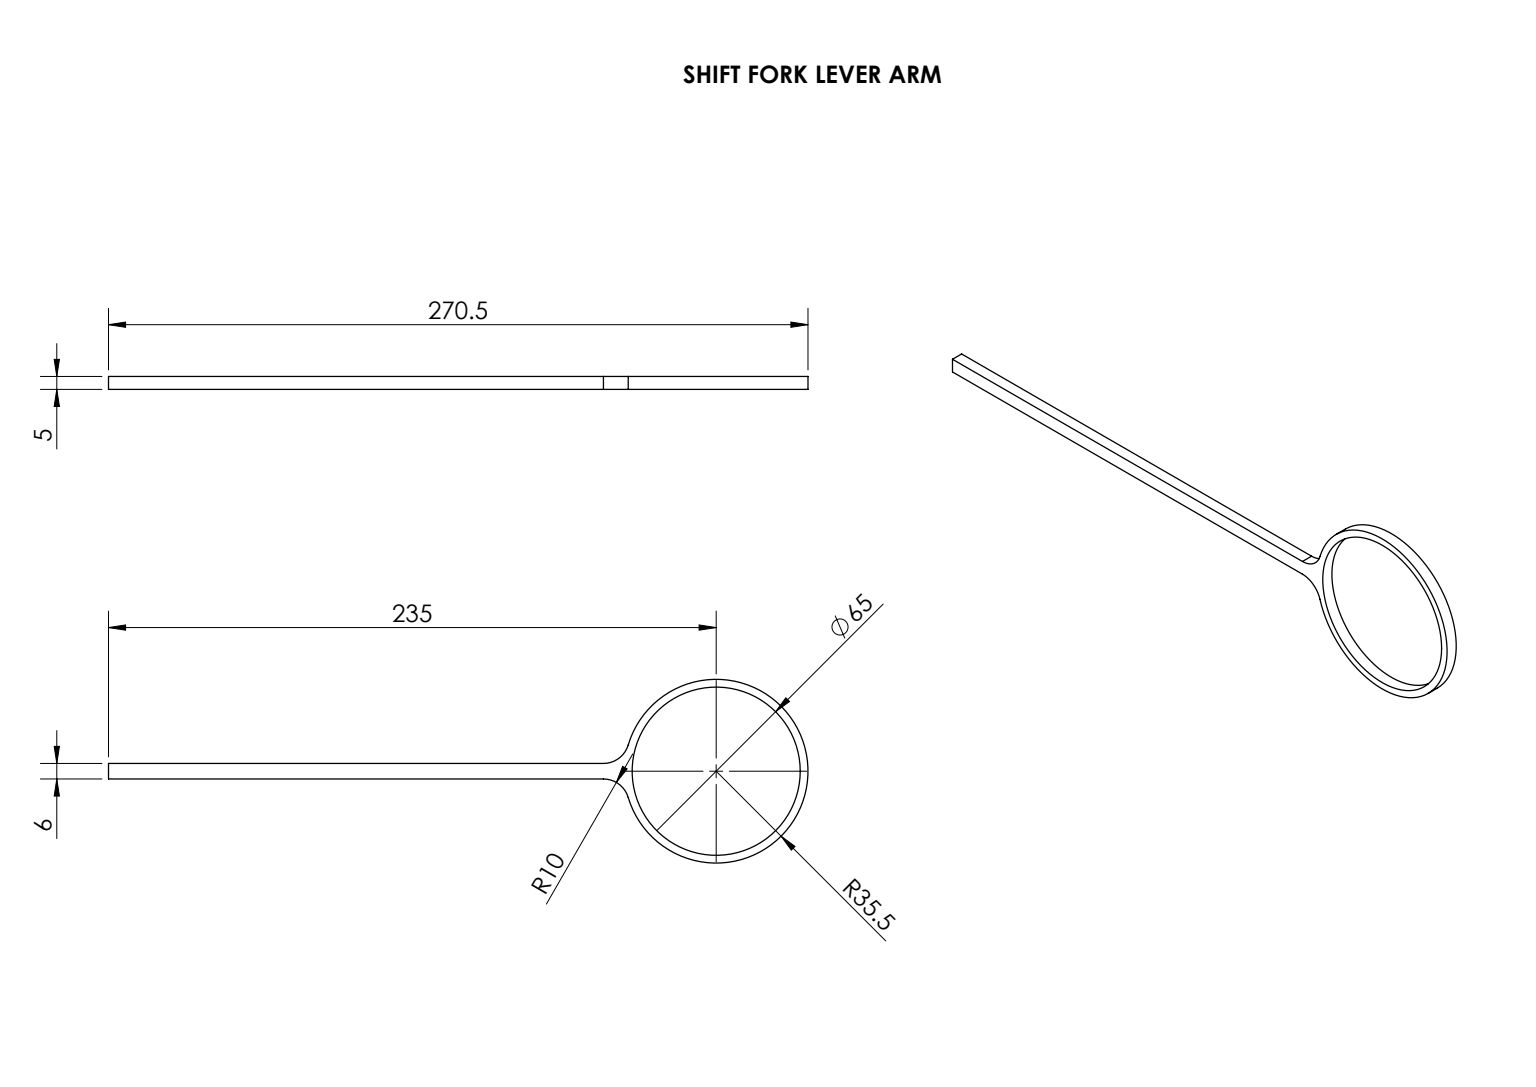
ISO-10303-21;
HEADER;
FILE_DESCRIPTION (('STEP AP214'),
    '1' );
FILE_NAME ('Shift Fork Lever Arm.step',
    '2026-09-30T12:41:04',
    ( '' ),
    ( '' ),
    'SwSTEP 2.0',
    'SolidWorks 2026',
    '' );
FILE_SCHEMA (( 'AUTOMOTIVE_DESIGN' ));
ENDSEC;

DATA;
#251=EDGE_CURVE ( 'NONE', #37160, #31484, #24741, .T. ) ;
#287=AXIS2_PLACEMENT_3D ( 'NONE', #20110, #9559, #24504 ) ;
#332=LINE ( 'NONE', #22378, #45772 ) ;
#605=ADVANCED_BREP_SHAPE_REPRESENTATION ( '', ( #3244, #11636 ), #6986 ) ;
#623=DIRECTION ( 'NONE',  ( 0.000000000000000000, 0.000000000000000000, 1.000000000000000000 ) ) ;
#1121=PRODUCT_DEFINITION ( 'UNKNOWN', '', #32690, #14935 ) ;
#1167=DIRECTION ( 'NONE',  ( 1.000000000000000000, 0.000000000000000000, 0.000000000000000000 ) ) ;
#1414=ORIENTED_EDGE ( 'NONE', *, *, #47268, .F. ) ;
#1530=EDGE_CURVE ( 'NONE', #31484, #24326, #4202, .T. ) ;
#1531=CARTESIAN_POINT ( 'NONE',  ( -43.60332556124591719, -117.0000000000000000, -2.500000000000002220 ) ) ;
#1603=ORIENTED_EDGE ( 'NONE', *, *, #35461, .T. ) ;
#1694=FILL_AREA_STYLE_COLOUR ( '', #30434 ) ;
#1768=VECTOR ( 'NONE', #29838, 1000.000000000000000 ) ;
#1821=EDGE_LOOP ( 'NONE', ( #25451, #11030, #4966, #38289 ) ) ;
#1945=( NAMED_UNIT ( * ) SI_UNIT ( $, .STERADIAN. ) SOLID_ANGLE_UNIT ( ) );
#2151=DIRECTION ( 'NONE',  ( -1.000000000000000000, 0.000000000000000000, 0.000000000000000000 ) ) ;
#2172=DIRECTION ( 'NONE',  ( 1.000000000000000000, 0.000000000000000000, 0.000000000000000000 ) ) ;
#2540=DIRECTION ( 'NONE',  ( 1.000000000000000000, 0.000000000000000000, 0.000000000000000000 ) ) ;
#2824=ADVANCED_FACE ( 'NONE', ( #8419 ), #23345, .F. ) ;
#2951=DIRECTION ( 'NONE',  ( 0.000000000000000000, 0.000000000000000000, 1.000000000000000000 ) ) ;
#3244=MANIFOLD_SOLID_BREP ( 'Fillet1', #6745 ) ;
#3247=VECTOR ( 'NONE', #47516, 1000.000000000000000 ) ;
#3362=ORIENTED_EDGE ( 'NONE', *, *, #41369, .F. ) ;
#3400=CARTESIAN_POINT ( 'NONE',  ( -235.0000123116479926, -117.0000000000000142, 2.500000000000000000 ) ) ;
#3500=ORIENTED_EDGE ( 'NONE', *, *, #6790, .F. ) ;
#3532=DIRECTION ( 'NONE',  ( -0.000000000000000000, -0.000000000000000000, -1.000000000000000000 ) ) ;
#3667=DIRECTION ( 'NONE',  ( 1.000000000000000000, 0.000000000000000000, 0.000000000000000000 ) ) ;
#3690=VERTEX_POINT ( 'NONE', #9677 ) ;
#3885=CARTESIAN_POINT ( 'NONE',  ( -43.60332556124591008, -133.0000000000000000, 2.500000000000002220 ) ) ;
#3916=FACE_OUTER_BOUND ( 'NONE', #19929, .T. ) ;
#4202=LINE ( 'NONE', #30155, #45519 ) ;
#4484=CARTESIAN_POINT ( 'NONE',  ( -35.37301231164799731, -117.0000000000000000, 2.500000000000000000 ) ) ;
#4520=ORIENTED_EDGE ( 'NONE', *, *, #32367, .F. ) ;
#4521=CARTESIAN_POINT ( 'NONE',  ( -35.37301231164799731, -123.0000000000000142, 2.500000000000000000 ) ) ;
#4650=VERTEX_POINT ( 'NONE', #6360 ) ;
#4684=FACE_BOUND ( 'NONE', #4938, .T. ) ;
#4787=ORIENTED_EDGE ( 'NONE', *, *, #19891, .F. ) ;
#4938=EDGE_LOOP ( 'NONE', ( #16511, #37210 ) ) ;
#4966=ORIENTED_EDGE ( 'NONE', *, *, #11266, .T. ) ;
#5358=( NAMED_UNIT ( * ) PLANE_ANGLE_UNIT ( ) SI_UNIT ( $, .RADIAN. ) );
#5684=ORIENTED_EDGE ( 'NONE', *, *, #1530, .F. ) ;
#5751=ORIENTED_EDGE ( 'NONE', *, *, #29832, .T. ) ;
#6138=FACE_OUTER_BOUND ( 'NONE', #42443, .T. ) ;
#6195=PRODUCT ( 'Shift Fork Lever Arm', 'Shift Fork Lever Arm', '', ( #34306 ) ) ;
#6360=CARTESIAN_POINT ( 'NONE',  ( -34.02017708624680381, -130.1428571428571388, 2.500000000000000000 ) ) ;
#6380=CARTESIAN_POINT ( 'NONE',  ( -235.0000123116479926, -123.0000000000000284, 2.500000000000000000 ) ) ;
#6513=ORIENTED_EDGE ( 'NONE', *, *, #11266, .F. ) ;
#6619=DIRECTION ( 'NONE',  ( 0.000000000000000000, 0.000000000000000000, 1.000000000000000000 ) ) ;
#6701=ADVANCED_FACE ( 'NONE', ( #47322 ), #17918, .F. ) ;
#6745=CLOSED_SHELL ( 'NONE', ( #35945, #26592, #34256, #14741, #7793, #6701, #7128, #14982, #2824, #10559 ) ) ;
#6790=EDGE_CURVE ( 'NONE', #4650, #23089, #28936, .T. ) ;
#6884=VERTEX_POINT ( 'NONE', #22808 ) ;
#6887=CARTESIAN_POINT ( 'NONE',  ( 0.000000000000000000, -120.0000000000000000, 2.500000000000000000 ) ) ;
#6918=DIRECTION ( 'NONE',  ( 1.000000000000000000, 1.390371824233641368E-16, 0.000000000000000000 ) ) ;
#6986=( GEOMETRIC_REPRESENTATION_CONTEXT ( 3 ) GLOBAL_UNCERTAINTY_ASSIGNED_CONTEXT ( ( #45275 ) ) GLOBAL_UNIT_ASSIGNED_CONTEXT ( ( #16379, #12963, #1945 ) ) REPRESENTATION_CONTEXT ( 'NONE', 'WORKASPACE' ) );
#7063=VERTEX_POINT ( 'NONE', #32091 ) ;
#7128=ADVANCED_FACE ( 'NONE', ( #6138 ), #40156, .F. ) ;
#7647=CARTESIAN_POINT ( 'NONE',  ( -43.60332556124591008, -133.0000000000000000, -2.500000000000002220 ) ) ;
#7699=LINE ( 'NONE', #4521, #35749 ) ;
#7793=ADVANCED_FACE ( 'NONE', ( #14292, #29224 ), #36086, .T. ) ;
#7877=DIRECTION ( 'NONE',  ( 1.000000000000000000, 0.000000000000000000, 0.000000000000000000 ) ) ;
#8419=FACE_OUTER_BOUND ( 'NONE', #20142, .T. ) ;
#9028=SURFACE_STYLE_FILL_AREA ( #9744 ) ;
#9258=DIRECTION ( 'NONE',  ( 1.000000000000000000, 0.000000000000000000, 0.000000000000000000 ) ) ;
#9269=SURFACE_STYLE_FILL_AREA ( #39382 ) ;
#9453=AXIS2_PLACEMENT_3D ( 'NONE', #3885, #30815, #45740 ) ;
#9498=MECHANICAL_DESIGN_GEOMETRIC_PRESENTATION_REPRESENTATION('',(#14180),#43704);
#9504=PRESENTATION_STYLE_ASSIGNMENT (( #28351 ) ) ;
#9509=AXIS2_PLACEMENT_3D ( 'NONE', #39245, #35084, #46346 ) ;
#9559=DIRECTION ( 'NONE',  ( 0.000000000000000000, 0.000000000000000000, -1.000000000000000000 ) ) ;
#9677=CARTESIAN_POINT ( 'NONE',  ( -34.02017708624681092, -109.8571428571428470, -2.500000000000000000 ) ) ;
#9744=FILL_AREA_STYLE ('',( #39371 ) ) ;
#9752=( NAMED_UNIT ( * ) PLANE_ANGLE_UNIT ( ) SI_UNIT ( $, .RADIAN. ) );
#10079=CARTESIAN_POINT ( 'NONE',  ( -235.0000123116479926, -123.0000000000000284, 2.500000000000000000 ) ) ;
#10171=ORIENTED_EDGE ( 'NONE', *, *, #27871, .F. ) ;
#10234=FACE_OUTER_BOUND ( 'NONE', #19948, .T. ) ;
#10261=ORIENTED_EDGE ( 'NONE', *, *, #37960, .T. ) ;
#10299=ORIENTED_EDGE ( 'NONE', *, *, #1530, .T. ) ;
#10338=DIRECTION ( 'NONE',  ( 1.390371824233641368E-16, -1.000000000000000000, 0.000000000000000000 ) ) ;
#10559=ADVANCED_FACE ( 'NONE', ( #44108 ), #43865, .F. ) ;
#10633=EDGE_LOOP ( 'NONE', ( #6513, #1603, #27465, #14120, #33764, #29148 ) ) ;
#11030=ORIENTED_EDGE ( 'NONE', *, *, #6790, .T. ) ;
#11266=EDGE_CURVE ( 'NONE', #23089, #3690, #38838, .T. ) ;
#11419=CARTESIAN_POINT ( 'NONE',  ( -34.02017708624681092, -109.8571428571428470, 102.9091629284897493 ) ) ;
#11514=UNCERTAINTY_MEASURE_WITH_UNIT (LENGTH_MEASURE( 1.000000000000000082E-05 ), #31811, 'distance_accuracy_value', 'NONE');
#11636=AXIS2_PLACEMENT_3D ( 'NONE', #13959, #6619, #3667 ) ;
#12029=ORIENTED_EDGE ( 'NONE', *, *, #40303, .T. ) ;
#12829=LINE ( 'NONE', #24567, #18286 ) ;
#12963=( NAMED_UNIT ( * ) PLANE_ANGLE_UNIT ( ) SI_UNIT ( $, .RADIAN. ) );
#13182=SURFACE_SIDE_STYLE ('',( #9028 ) ) ;
#13211=EDGE_CURVE ( 'NONE', #30765, #19987, #36238, .T. ) ;
#13759=DIRECTION ( 'NONE',  ( -0.000000000000000000, -1.000000000000000000, -0.000000000000000000 ) ) ;
#13955=AXIS2_PLACEMENT_3D ( 'NONE', #28576, #43510, #2151 ) ;
#13959=CARTESIAN_POINT ( 'NONE',  ( 0.000000000000000000, 0.000000000000000000, 0.000000000000000000 ) ) ;
#14013=STYLED_ITEM ( 'NONE', ( #9504 ), #605 ) ;
#14120=ORIENTED_EDGE ( 'NONE', *, *, #17340, .F. ) ;
#14148=APPLICATION_CONTEXT ( 'automotive_design' ) ;
#14180=STYLED_ITEM ( 'NONE', ( #20512 ), #3244 ) ;
#14277=ORIENTED_EDGE ( 'NONE', *, *, #41080, .T. ) ;
#14292=FACE_BOUND ( 'NONE', #35647, .T. ) ;
#14311=CARTESIAN_POINT ( 'NONE',  ( 0.000000000000000000, -120.0000000000000000, 102.9091629284897493 ) ) ;
#14741=ADVANCED_FACE ( 'NONE', ( #3916 ), #38418, .F. ) ;
#14774=CARTESIAN_POINT ( 'NONE',  ( -235.0000123116479926, -123.0000000000000284, -2.500000000000000000 ) ) ;
#14935=PRODUCT_DEFINITION_CONTEXT ( 'detailed design', #25696, 'design' ) ;
#14982=ADVANCED_FACE ( 'NONE', ( #10234 ), #17816, .F. ) ;
#15188=DIRECTION ( 'NONE',  ( -0.000000000000000000, -0.000000000000000000, -1.000000000000000000 ) ) ;
#15284=DIRECTION ( 'NONE',  ( -0.000000000000000000, -1.000000000000000000, -0.000000000000000000 ) ) ;
#15715=ORIENTED_EDGE ( 'NONE', *, *, #17340, .T. ) ;
#15735=EDGE_CURVE ( 'NONE', #22256, #24326, #17476, .T. ) ;
#15973=EDGE_CURVE ( 'NONE', #24326, #22256, #31632, .T. ) ;
#16126=AXIS2_PLACEMENT_3D ( 'NONE', #36532, #10338, #6918 ) ;
#16221=ORIENTED_EDGE ( 'NONE', *, *, #33483, .F. ) ;
#16379=( LENGTH_UNIT ( ) NAMED_UNIT ( * ) SI_UNIT ( .MILLI., .METRE. ) );
#16511=ORIENTED_EDGE ( 'NONE', *, *, #15973, .T. ) ;
#16637=AXIS2_PLACEMENT_3D ( 'NONE', #46060, #42140, #34536 ) ;
#17183=DIRECTION ( 'NONE',  ( -0.000000000000000000, -0.000000000000000000, -1.000000000000000000 ) ) ;
#17340=EDGE_CURVE ( 'NONE', #21962, #40162, #32360, .T. ) ;
#17476=CIRCLE ( 'NONE', #33894, 32.50000000000000000 ) ;
#17811=MECHANICAL_DESIGN_GEOMETRIC_PRESENTATION_REPRESENTATION('',(#14013),#30340);
#17816=PLANE ( 'NONE',  #37872 ) ;
#17868=UNCERTAINTY_MEASURE_WITH_UNIT (LENGTH_MEASURE( 1.000000000000000082E-05 ), #38906, 'distance_accuracy_value', 'NONE');
#17918=PLANE ( 'NONE',  #16126 ) ;
#18286=VECTOR ( 'NONE', #35328, 1000.000000000000000 ) ;
#18372=AXIS2_PLACEMENT_3D ( 'NONE', #6380, #21288, #35984 ) ;
#18383=DIRECTION ( 'NONE',  ( 0.000000000000000000, 0.000000000000000000, 1.000000000000000000 ) ) ;
#18497=CARTESIAN_POINT ( 'NONE',  ( -35.37301231164799731, -123.0000000000000142, -2.500000000000000000 ) ) ;
#18605=CARTESIAN_POINT ( 'NONE',  ( 0.000000000000000000, -120.0000000000000000, 102.9091629284897493 ) ) ;
#19142=EDGE_CURVE ( 'NONE', #22787, #4650, #24311, .T. ) ;
#19322=DIRECTION ( 'NONE',  ( -1.000000000000000000, 0.000000000000000000, 0.000000000000000000 ) ) ;
#19369=CIRCLE ( 'NONE', #44391, 10.00000000000000178 ) ;
#19587=DIRECTION ( 'NONE',  ( 0.000000000000000000, 0.000000000000000000, 1.000000000000000000 ) ) ;
#19891=EDGE_CURVE ( 'NONE', #44730, #3690, #43069, .T. ) ;
#19929=EDGE_LOOP ( 'NONE', ( #25882, #21207, #10299, #47041 ) ) ;
#19948=EDGE_LOOP ( 'NONE', ( #10261, #41037, #1414, #28073 ) ) ;
#19987=VERTEX_POINT ( 'NONE', #37481 ) ;
#20110=CARTESIAN_POINT ( 'NONE',  ( -43.60332556124591719, -107.0000000000000000, 2.500000000000002220 ) ) ;
#20142=EDGE_LOOP ( 'NONE', ( #24294, #16221, #37606, #3500 ) ) ;
#20512=PRESENTATION_STYLE_ASSIGNMENT (( #24430 ) ) ;
#20767=( NAMED_UNIT ( * ) SI_UNIT ( $, .STERADIAN. ) SOLID_ANGLE_UNIT ( ) );
#20775=( NAMED_UNIT ( * ) SI_UNIT ( $, .STERADIAN. ) SOLID_ANGLE_UNIT ( ) );
#20925=CARTESIAN_POINT ( 'NONE',  ( 0.000000000000000000, -89.50000000000000000, 2.500000000000000000 ) ) ;
#21207=ORIENTED_EDGE ( 'NONE', *, *, #251, .T. ) ;
#21288=DIRECTION ( 'NONE',  ( 1.000000000000000000, 0.000000000000000000, 0.000000000000000000 ) ) ;
#21656=CYLINDRICAL_SURFACE ( 'NONE', #40105, 35.50000000000001421 ) ;
#21675=EDGE_CURVE ( 'NONE', #6884, #21962, #36928, .T. ) ;
#21807=LINE ( 'NONE', #10079, #3247 ) ;
#21962=VERTEX_POINT ( 'NONE', #47650 ) ;
#22256=VERTEX_POINT ( 'NONE', #41781 ) ;
#22378=CARTESIAN_POINT ( 'NONE',  ( -235.0000123116479926, -123.0000000000000284, 2.500000000000000000 ) ) ;
#22574=DIRECTION ( 'NONE',  ( 0.000000000000000000, 0.000000000000000000, 1.000000000000000000 ) ) ;
#22706=EDGE_CURVE ( 'NONE', #44730, #21962, #12829, .T. ) ;
#22787=VERTEX_POINT ( 'NONE', #36052 ) ;
#22808=CARTESIAN_POINT ( 'NONE',  ( -235.0000123116479926, -117.0000000000000142, 2.500000000000000000 ) ) ;
#23089=VERTEX_POINT ( 'NONE', #42141 ) ;
#23345=CYLINDRICAL_SURFACE ( 'NONE', #9509, 10.00000000000000178 ) ;
#23764=PLANE ( 'NONE',  #47403 ) ;
#24294=ORIENTED_EDGE ( 'NONE', *, *, #19142, .F. ) ;
#24311=CIRCLE ( 'NONE', #9453, 10.00000000000000178 ) ;
#24326=VERTEX_POINT ( 'NONE', #39157 ) ;
#24430=SURFACE_STYLE_USAGE ( .BOTH. , #13182 ) ;
#24504=DIRECTION ( 'NONE',  ( 1.000000000000000000, 1.387778780781445478E-15, 0.000000000000000000 ) ) ;
#24567=CARTESIAN_POINT ( 'NONE',  ( -35.37301231164799731, -117.0000000000000000, -2.500000000000000000 ) ) ;
#24741=CIRCLE ( 'NONE', #29316, 32.50000000000000000 ) ;
#24983=VECTOR ( 'NONE', #38075, 1000.000000000000000 ) ;
#25451=ORIENTED_EDGE ( 'NONE', *, *, #29832, .F. ) ;
#25499=DIRECTION ( 'NONE',  ( -1.000000000000000000, 0.000000000000000000, 0.000000000000000000 ) ) ;
#25583=ORIENTED_EDGE ( 'NONE', *, *, #22706, .T. ) ;
#25696=APPLICATION_CONTEXT ( 'automotive_design' ) ;
#25882=ORIENTED_EDGE ( 'NONE', *, *, #41080, .F. ) ;
#25889=AXIS2_PLACEMENT_3D ( 'NONE', #27128, #38873, #1167 ) ;
#26551=DIRECTION ( 'NONE',  ( 1.000000000000000000, 6.951859121168206841E-17, -0.000000000000000000 ) ) ;
#26592=ADVANCED_FACE ( 'NONE', ( #40272 ), #21656, .T. ) ;
#26972=FACE_OUTER_BOUND ( 'NONE', #10633, .T. ) ;
#27128=CARTESIAN_POINT ( 'NONE',  ( 0.000000000000000000, -120.0000000000000000, 2.500000000000000000 ) ) ;
#27193=ORIENTED_EDGE ( 'NONE', *, *, #40473, .T. ) ;
#27203=EDGE_LOOP ( 'NONE', ( #31989, #14277, #33908, #5684 ) ) ;
#27228=SHAPE_DEFINITION_REPRESENTATION ( #43706, #40966 ) ;
#27465=ORIENTED_EDGE ( 'NONE', *, *, #37960, .F. ) ;
#27871=EDGE_CURVE ( 'NONE', #3690, #30765, #44935, .T. ) ;
#27892=CARTESIAN_POINT ( 'NONE',  ( 0.000000000000000000, -120.0000000000000000, -2.500000000000000000 ) ) ;
#28051=CARTESIAN_POINT ( 'NONE',  ( -43.60332556124591008, -123.0000000000000142, 2.500000000000002220 ) ) ;
#28073=ORIENTED_EDGE ( 'NONE', *, *, #41835, .T. ) ;
#28351=SURFACE_STYLE_USAGE ( .BOTH. , #47200 ) ;
#28371=LINE ( 'NONE', #47220, #43825 ) ;
#28469=AXIS2_PLACEMENT_3D ( 'NONE', #35702, #46730, #2172 ) ;
#28513=DIRECTION ( 'NONE',  ( 0.000000000000000000, -0.000000000000000000, 1.000000000000000000 ) ) ;
#28576=CARTESIAN_POINT ( 'NONE',  ( 0.000000000000000000, -120.0000000000000000, 102.9091629284897493 ) ) ;
#28897=DIRECTION ( 'NONE',  ( 1.000000000000000000, 0.000000000000000000, 0.000000000000000000 ) ) ;
#28936=LINE ( 'NONE', #32392, #38018 ) ;
#29140=CARTESIAN_POINT ( 'NONE',  ( -43.60332556124591719, -107.0000000000000000, -2.500000000000002220 ) ) ;
#29148=ORIENTED_EDGE ( 'NONE', *, *, #19891, .T. ) ;
#29179=DIRECTION ( 'NONE',  ( -0.000000000000000000, -0.000000000000000000, -1.000000000000000000 ) ) ;
#29224=FACE_OUTER_BOUND ( 'NONE', #40265, .T. ) ;
#29316=AXIS2_PLACEMENT_3D ( 'NONE', #6887, #18383, #48245 ) ;
#29396=DIRECTION ( 'NONE',  ( 0.000000000000000000, 0.000000000000000000, 1.000000000000000000 ) ) ;
#29427=CARTESIAN_POINT ( 'NONE',  ( -43.60332556124591719, -107.0000000000000000, 102.9091629284897493 ) ) ;
#29832=EDGE_CURVE ( 'NONE', #4650, #30765, #42457, .T. ) ;
#29838=DIRECTION ( 'NONE',  ( -0.000000000000000000, -0.000000000000000000, -1.000000000000000000 ) ) ;
#30007=VECTOR ( 'NONE', #46077, 1000.000000000000000 ) ;
#30155=CARTESIAN_POINT ( 'NONE',  ( -32.50000000000000000, -120.0000000000000000, 102.9091629284897493 ) ) ;
#30340=( GEOMETRIC_REPRESENTATION_CONTEXT ( 3 ) GLOBAL_UNCERTAINTY_ASSIGNED_CONTEXT ( ( #17868 ) ) GLOBAL_UNIT_ASSIGNED_CONTEXT ( ( #38906, #9752, #20775 ) ) REPRESENTATION_CONTEXT ( 'NONE', 'WORKASPACE' ) );
#30434=COLOUR_RGB ( '', 0.31764706, 0.68627451, 0.89019608) ;
#30583=CARTESIAN_POINT ( 'NONE',  ( -32.50000000000000000, -120.0000000000000000, 2.500000000000000000 ) ) ;
#30765=VERTEX_POINT ( 'NONE', #31203 ) ;
#30783=ORIENTED_EDGE ( 'NONE', *, *, #40473, .F. ) ;
#30815=DIRECTION ( 'NONE',  ( 0.000000000000000000, 0.000000000000000000, -1.000000000000000000 ) ) ;
#31158=LINE ( 'NONE', #1531, #30007 ) ;
#31203=CARTESIAN_POINT ( 'NONE',  ( -34.02017708624680381, -109.8571428571428470, 2.500000000000000000 ) ) ;
#31484=VERTEX_POINT ( 'NONE', #30583 ) ;
#31535=ORIENTED_EDGE ( 'NONE', *, *, #19142, .T. ) ;
#31632=CIRCLE ( 'NONE', #28469, 32.50000000000000000 ) ;
#31741=LINE ( 'NONE', #28051, #35634 ) ;
#31811=( LENGTH_UNIT ( ) NAMED_UNIT ( * ) SI_UNIT ( .MILLI., .METRE. ) );
#31989=ORIENTED_EDGE ( 'NONE', *, *, #41369, .T. ) ;
#32091=CARTESIAN_POINT ( 'NONE',  ( -235.0000123116479926, -123.0000000000000284, 2.500000000000000000 ) ) ;
#32360=LINE ( 'NONE', #40651, #44674 ) ;
#32367=EDGE_CURVE ( 'NONE', #6884, #7063, #332, .T. ) ;
#32392=CARTESIAN_POINT ( 'NONE',  ( -34.02017708624681092, -130.1428571428571388, 102.9091629284897493 ) ) ;
#32690=PRODUCT_DEFINITION_FORMATION_WITH_SPECIFIED_SOURCE ( 'ANY', '', #6195, .NOT_KNOWN. ) ;
#33146=AXIS2_PLACEMENT_3D ( 'NONE', #18605, #15188, #19322 ) ;
#33241=CARTESIAN_POINT ( 'NONE',  ( -35.37301231164799731, -123.0000000000000142, 2.500000000000000000 ) ) ;
#33483=EDGE_CURVE ( 'NONE', #46110, #22787, #31741, .T. ) ;
#33764=ORIENTED_EDGE ( 'NONE', *, *, #22706, .F. ) ;
#33894=AXIS2_PLACEMENT_3D ( 'NONE', #44323, #29396, #28897 ) ;
#33908=ORIENTED_EDGE ( 'NONE', *, *, #15973, .F. ) ;
#34253=CARTESIAN_POINT ( 'NONE',  ( 32.50000000000000000, -120.0000000000000000, 2.500000000000000000 ) ) ;
#34256=ADVANCED_FACE ( 'NONE', ( #26972, #4684 ), #23764, .F. ) ;
#34282=CARTESIAN_POINT ( 'NONE',  ( -43.60332556124591719, -117.0000000000000000, -2.500000000000000000 ) ) ;
#34306=PRODUCT_CONTEXT ( 'NONE', #14148, 'mechanical' ) ;
#34536=DIRECTION ( 'NONE',  ( 1.000000000000000000, 0.000000000000000000, 0.000000000000000000 ) ) ;
#35020=CARTESIAN_POINT ( 'NONE',  ( 0.000000000000000000, -120.0000000000000000, -2.500000000000000000 ) ) ;
#35084=DIRECTION ( 'NONE',  ( -0.000000000000000000, -0.000000000000000000, -1.000000000000000000 ) ) ;
#35166=ORIENTED_EDGE ( 'NONE', *, *, #40303, .F. ) ;
#35269=CIRCLE ( 'NONE', #25889, 32.50000000000000000 ) ;
#35281=COLOUR_RGB ( '', 0.31764706, 0.68627451, 0.89019608) ;
#35328=DIRECTION ( 'NONE',  ( -1.000000000000000000, -1.390371824233641368E-16, 0.000000000000000000 ) ) ;
#35461=EDGE_CURVE ( 'NONE', #23089, #46110, #19369, .T. ) ;
#35634=VECTOR ( 'NONE', #42978, 1000.000000000000000 ) ;
#35647=EDGE_LOOP ( 'NONE', ( #3362, #36980 ) ) ;
#35678=CYLINDRICAL_SURFACE ( 'NONE', #13955, 32.50000000000000000 ) ;
#35702=CARTESIAN_POINT ( 'NONE',  ( 0.000000000000000000, -120.0000000000000000, -2.500000000000000000 ) ) ;
#35749=VECTOR ( 'NONE', #26551, 1000.000000000000000 ) ;
#35945=ADVANCED_FACE ( 'NONE', ( #47637 ), #35678, .F. ) ;
#35984=DIRECTION ( 'NONE',  ( 0.000000000000000000, 0.000000000000000000, -1.000000000000000000 ) ) ;
#36005=DIRECTION ( 'NONE',  ( 1.000000000000000000, 0.000000000000000000, 0.000000000000000000 ) ) ;
#36052=CARTESIAN_POINT ( 'NONE',  ( -43.60332556124591008, -123.0000000000000142, 2.500000000000000000 ) ) ;
#36086=PLANE ( 'NONE',  #37443 ) ;
#36238=CIRCLE ( 'NONE', #287, 10.00000000000000178 ) ;
#36271=ORIENTED_EDGE ( 'NONE', *, *, #13211, .F. ) ;
#36532=CARTESIAN_POINT ( 'NONE',  ( -35.37301231164799731, -117.0000000000000000, 2.500000000000000000 ) ) ;
#36578=DIRECTION ( 'NONE',  ( -1.000000000000000000, 0.000000000000000000, 0.000000000000000000 ) ) ;
#36850=EDGE_LOOP ( 'NONE', ( #36271, #10171, #4787, #30783 ) ) ;
#36928=LINE ( 'NONE', #3400, #1768 ) ;
#36980=ORIENTED_EDGE ( 'NONE', *, *, #251, .F. ) ;
#37160=VERTEX_POINT ( 'NONE', #34253 ) ;
#37210=ORIENTED_EDGE ( 'NONE', *, *, #15735, .T. ) ;
#37443=AXIS2_PLACEMENT_3D ( 'NONE', #20925, #28513, #2540 ) ;
#37481=CARTESIAN_POINT ( 'NONE',  ( -43.60332556124591719, -117.0000000000000000, 2.500000000000000000 ) ) ;
#37606=ORIENTED_EDGE ( 'NONE', *, *, #35461, .F. ) ;
#37872=AXIS2_PLACEMENT_3D ( 'NONE', #33241, #44496, #47669 ) ;
#37960=EDGE_CURVE ( 'NONE', #40162, #46110, #40771, .T. ) ;
#38018=VECTOR ( 'NONE', #29179, 1000.000000000000000 ) ;
#38075=DIRECTION ( 'NONE',  ( 1.000000000000000000, 6.951859121168206841E-17, -0.000000000000000000 ) ) ;
#38250=LINE ( 'NONE', #4484, #39413 ) ;
#38289=ORIENTED_EDGE ( 'NONE', *, *, #27871, .T. ) ;
#38418=CYLINDRICAL_SURFACE ( 'NONE', #33146, 32.50000000000000000 ) ;
#38751=ORIENTED_EDGE ( 'NONE', *, *, #47268, .T. ) ;
#38838=CIRCLE ( 'NONE', #45850, 35.50000000000001421 ) ;
#38873=DIRECTION ( 'NONE',  ( 0.000000000000000000, 0.000000000000000000, 1.000000000000000000 ) ) ;
#38906=( LENGTH_UNIT ( ) NAMED_UNIT ( * ) SI_UNIT ( .MILLI., .METRE. ) );
#39157=CARTESIAN_POINT ( 'NONE',  ( -32.50000000000000000, -120.0000000000000000, -2.500000000000000000 ) ) ;
#39245=CARTESIAN_POINT ( 'NONE',  ( -43.60332556124591008, -133.0000000000000000, 102.9091629284897493 ) ) ;
#39371=FILL_AREA_STYLE_COLOUR ( '', #35281 ) ;
#39382=FILL_AREA_STYLE ('',( #1694 ) ) ;
#39413=VECTOR ( 'NONE', #44867, 1000.000000000000000 ) ;
#39716=ORIENTED_EDGE ( 'NONE', *, *, #13211, .T. ) ;
#39928=AXIS2_PLACEMENT_3D ( 'NONE', #29140, #2951, #36005 ) ;
#40105=AXIS2_PLACEMENT_3D ( 'NONE', #14311, #3532, #36578 ) ;
#40156=PLANE ( 'NONE',  #18372 ) ;
#40162=VERTEX_POINT ( 'NONE', #14774 ) ;
#40169=ORIENTED_EDGE ( 'NONE', *, *, #41835, .F. ) ;
#40265=EDGE_LOOP ( 'NONE', ( #38751, #31535, #5751, #39716, #12029, #45250 ) ) ;
#40272=FACE_OUTER_BOUND ( 'NONE', #1821, .T. ) ;
#40303=EDGE_CURVE ( 'NONE', #19987, #6884, #38250, .T. ) ;
#40473=EDGE_CURVE ( 'NONE', #19987, #44730, #31158, .T. ) ;
#40651=CARTESIAN_POINT ( 'NONE',  ( -235.0000123116479926, -123.0000000000000284, -2.500000000000000000 ) ) ;
#40771=LINE ( 'NONE', #18497, #24983 ) ;
#40966=SHAPE_REPRESENTATION ( 'Shift Fork Lever Arm', ( #11636 ), #6986 ) ;
#41037=ORIENTED_EDGE ( 'NONE', *, *, #33483, .T. ) ;
#41080=EDGE_CURVE ( 'NONE', #37160, #22256, #28371, .T. ) ;
#41369=EDGE_CURVE ( 'NONE', #31484, #37160, #35269, .T. ) ;
#41547=ORIENTED_EDGE ( 'NONE', *, *, #21675, .T. ) ;
#41781=CARTESIAN_POINT ( 'NONE',  ( 32.50000000000000000, -120.0000000000000000, -2.500000000000000000 ) ) ;
#41835=EDGE_CURVE ( 'NONE', #7063, #40162, #21807, .T. ) ;
#42140=DIRECTION ( 'NONE',  ( -0.000000000000000000, -0.000000000000000000, 1.000000000000000000 ) ) ;
#42141=CARTESIAN_POINT ( 'NONE',  ( -34.02017708624681092, -130.1428571428571388, -2.500000000000000000 ) ) ;
#42363=DIRECTION ( 'NONE',  ( -0.000000000000000000, -0.000000000000000000, -1.000000000000000000 ) ) ;
#42372=DIRECTION ( 'NONE',  ( 1.000000000000000000, 0.000000000000000000, -0.000000000000000000 ) ) ;
#42443=EDGE_LOOP ( 'NONE', ( #15715, #40169, #4520, #41547 ) ) ;
#42457=CIRCLE ( 'NONE', #16637, 35.50000000000000711 ) ;
#42806=DIRECTION ( 'NONE',  ( 0.000000000000000000, 0.000000000000000000, 1.000000000000000000 ) ) ;
#42978=DIRECTION ( 'NONE',  ( 0.000000000000000000, 0.000000000000000000, 1.000000000000000000 ) ) ;
#43030=VECTOR ( 'NONE', #623, 1000.000000000000000 ) ;
#43042=AXIS2_PLACEMENT_3D ( 'NONE', #29427, #17183, #25499 ) ;
#43069=CIRCLE ( 'NONE', #39928, 10.00000000000000178 ) ;
#43510=DIRECTION ( 'NONE',  ( -0.000000000000000000, -0.000000000000000000, -1.000000000000000000 ) ) ;
#43704=( GEOMETRIC_REPRESENTATION_CONTEXT ( 3 ) GLOBAL_UNCERTAINTY_ASSIGNED_CONTEXT ( ( #11514 ) ) GLOBAL_UNIT_ASSIGNED_CONTEXT ( ( #31811, #5358, #20767 ) ) REPRESENTATION_CONTEXT ( 'NONE', 'WORKASPACE' ) );
#43706=PRODUCT_DEFINITION_SHAPE ( 'NONE', 'NONE',  #1121 ) ;
#43825=VECTOR ( 'NONE', #44020, 1000.000000000000000 ) ;
#43865=CYLINDRICAL_SURFACE ( 'NONE', #43042, 10.00000000000000178 ) ;
#44020=DIRECTION ( 'NONE',  ( -0.000000000000000000, -0.000000000000000000, -1.000000000000000000 ) ) ;
#44108=FACE_OUTER_BOUND ( 'NONE', #36850, .T. ) ;
#44323=CARTESIAN_POINT ( 'NONE',  ( 0.000000000000000000, -120.0000000000000000, -2.500000000000000000 ) ) ;
#44391=AXIS2_PLACEMENT_3D ( 'NONE', #7647, #22574, #7877 ) ;
#44496=DIRECTION ( 'NONE',  ( -6.951859121168206841E-17, 1.000000000000000000, 0.000000000000000000 ) ) ;
#44674=VECTOR ( 'NONE', #13759, 1000.000000000000000 ) ;
#44730=VERTEX_POINT ( 'NONE', #34282 ) ;
#44867=DIRECTION ( 'NONE',  ( -1.000000000000000000, -1.390371824233641368E-16, 0.000000000000000000 ) ) ;
#44935=LINE ( 'NONE', #11419, #43030 ) ;
#45250=ORIENTED_EDGE ( 'NONE', *, *, #32367, .T. ) ;
#45275=UNCERTAINTY_MEASURE_WITH_UNIT (LENGTH_MEASURE( 1.000000000000000082E-05 ), #16379, 'distance_accuracy_value', 'NONE');
#45391=EDGE_LOOP ( 'NONE', ( #35166, #27193, #25583, #46863 ) ) ;
#45519=VECTOR ( 'NONE', #42363, 1000.000000000000000 ) ;
#45740=DIRECTION ( 'NONE',  ( 1.000000000000000000, 0.000000000000000000, 0.000000000000000000 ) ) ;
#45772=VECTOR ( 'NONE', #15284, 1000.000000000000000 ) ;
#45850=AXIS2_PLACEMENT_3D ( 'NONE', #27892, #42806, #9258 ) ;
#46060=CARTESIAN_POINT ( 'NONE',  ( 0.000000000000000000, -120.0000000000000000, 2.500000000000000000 ) ) ;
#46077=DIRECTION ( 'NONE',  ( -0.000000000000000000, -0.000000000000000000, -1.000000000000000000 ) ) ;
#46110=VERTEX_POINT ( 'NONE', #46289 ) ;
#46289=CARTESIAN_POINT ( 'NONE',  ( -43.60332556124591008, -123.0000000000000142, -2.500000000000000000 ) ) ;
#46346=DIRECTION ( 'NONE',  ( -1.000000000000000000, 0.000000000000000000, 0.000000000000000000 ) ) ;
#46730=DIRECTION ( 'NONE',  ( 0.000000000000000000, 0.000000000000000000, 1.000000000000000000 ) ) ;
#46734=SHAPE_REPRESENTATION_RELATIONSHIP ( 'NONE' , 'NONE' ,  #40966, #605 ) ;
#46863=ORIENTED_EDGE ( 'NONE', *, *, #21675, .F. ) ;
#47041=ORIENTED_EDGE ( 'NONE', *, *, #15735, .F. ) ;
#47200=SURFACE_SIDE_STYLE ('',( #9269 ) ) ;
#47220=CARTESIAN_POINT ( 'NONE',  ( 32.50000000000000000, -120.0000000000000000, 102.9091629284897493 ) ) ;
#47268=EDGE_CURVE ( 'NONE', #7063, #22787, #7699, .T. ) ;
#47322=FACE_OUTER_BOUND ( 'NONE', #45391, .T. ) ;
#47403=AXIS2_PLACEMENT_3D ( 'NONE', #35020, #19587, #42372 ) ;
#47516=DIRECTION ( 'NONE',  ( -0.000000000000000000, -0.000000000000000000, -1.000000000000000000 ) ) ;
#47637=FACE_OUTER_BOUND ( 'NONE', #27203, .T. ) ;
#47650=CARTESIAN_POINT ( 'NONE',  ( -235.0000123116479926, -117.0000000000000142, -2.500000000000000000 ) ) ;
#47669=DIRECTION ( 'NONE',  ( -1.000000000000000000, -6.951859121168206841E-17, 0.000000000000000000 ) ) ;
#48245=DIRECTION ( 'NONE',  ( 1.000000000000000000, 0.000000000000000000, 0.000000000000000000 ) ) ;
ENDSEC;
END-ISO-10303-21;
